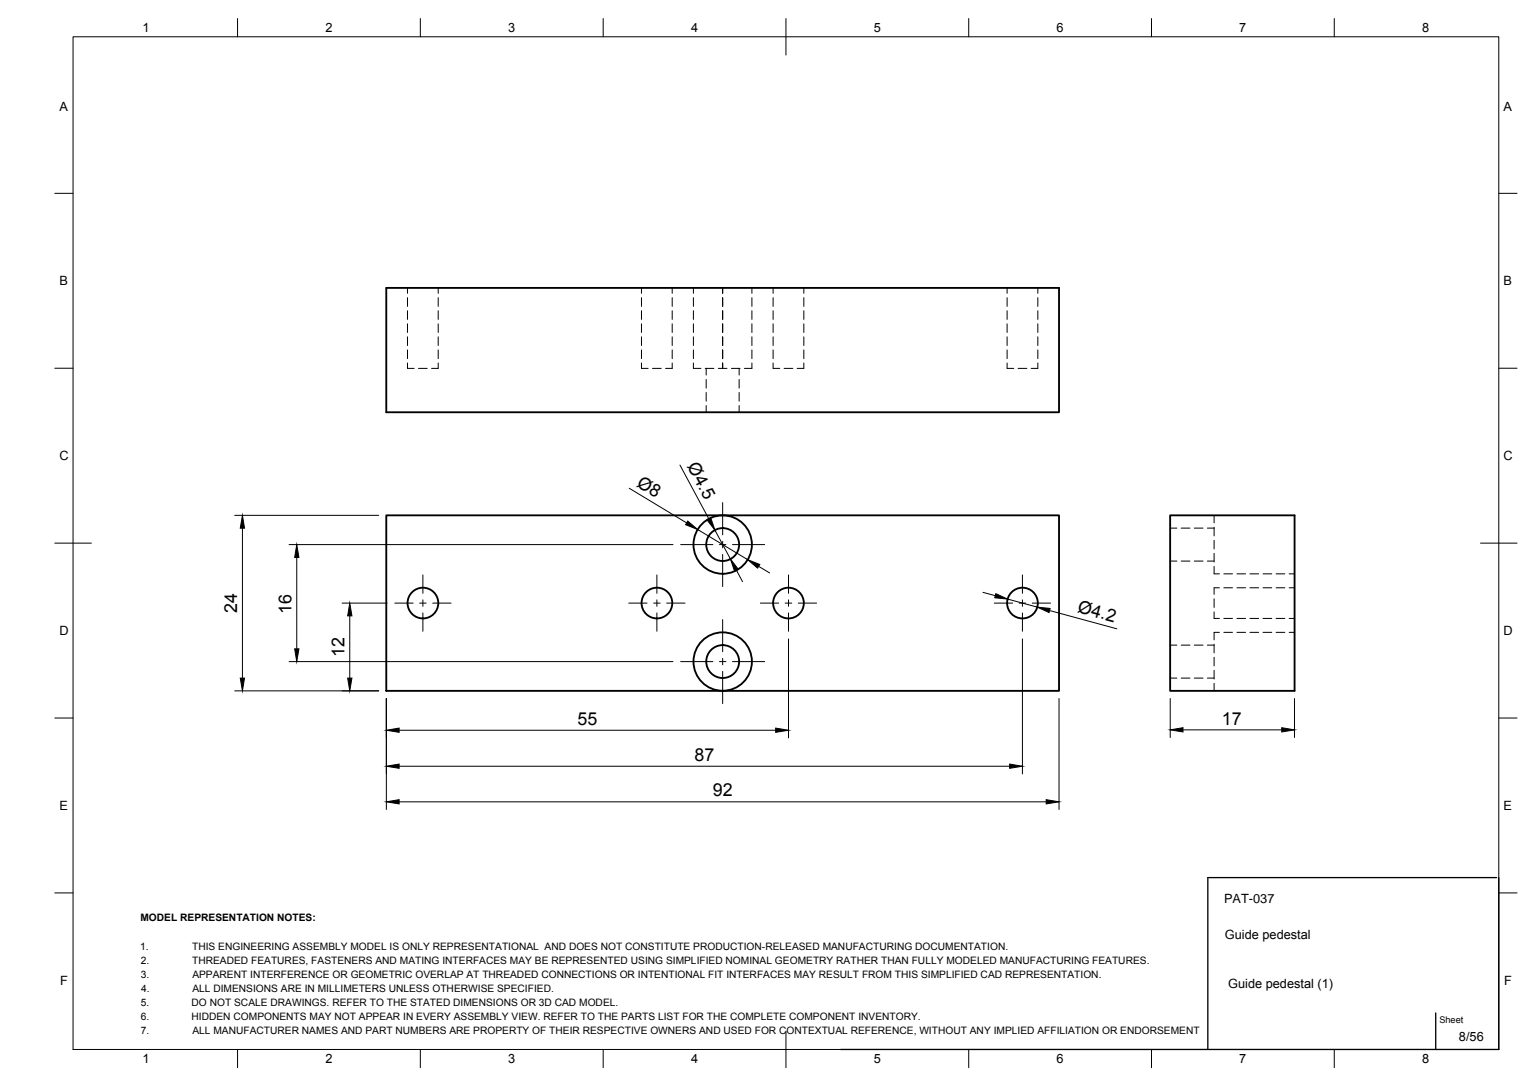
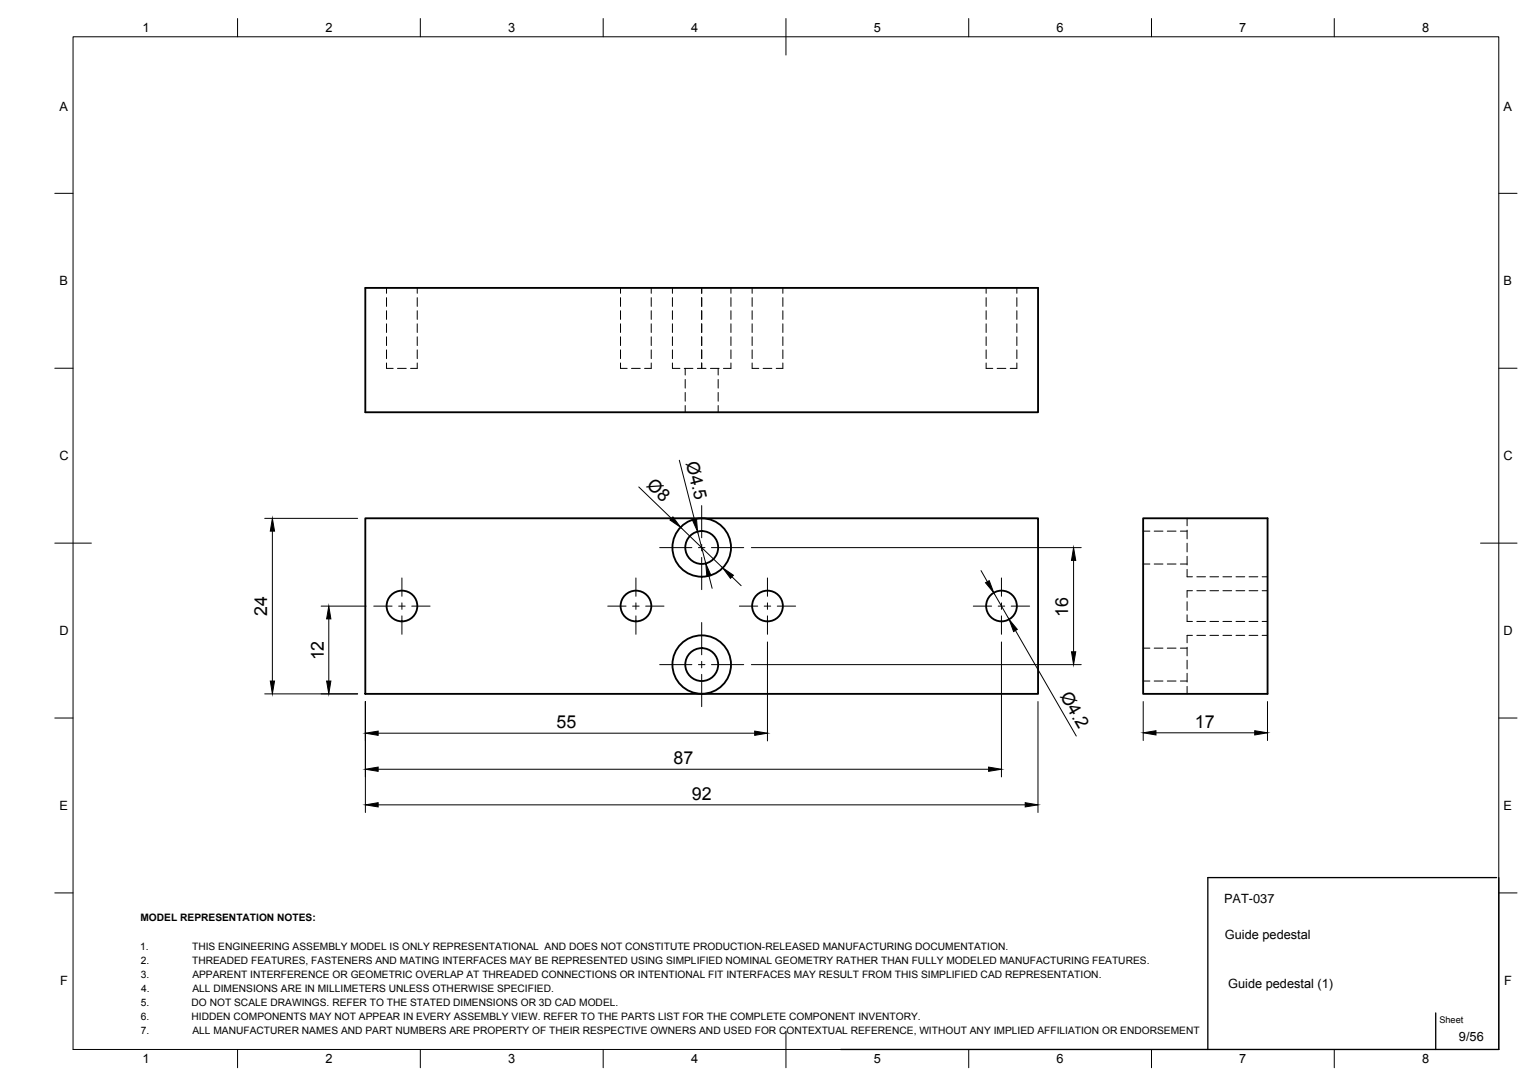
ISO-10303-21;
HEADER;
/* Generated by software containing ST-Developer
 * from STEP Tools, Inc. (www.steptools.com) 
 */

FILE_DESCRIPTION(
/* description */ ('Flywheel Crank-Slider'),
/* implementation_level */ '2;1');

FILE_NAME(
/* name */ 'Guide pedestal (1).step',
/* time_stamp */ '2026-10-28T03:23:13-07:00',
/* author */ (''),
/* organization */ (''),
/* preprocessor_version */ 'ST-DEVELOPER v20.2',
/* originating_system */ 'Autodesk Translation Framework v15.17.0.0',
/* authorisation */ '');

FILE_SCHEMA (('AUTOMOTIVE_DESIGN { 1 0 10303 214 3 1 1 }'));
ENDSEC;

DATA;
#10=MECHANICAL_DESIGN_GEOMETRIC_PRESENTATION_REPRESENTATION('',(#676),#17322);
#572=SHAPE_REPRESENTATION_RELATIONSHIP('SRR','None',#17568,#624);
#624=ADVANCED_BREP_SHAPE_REPRESENTATION('',(#737),#17272);
#676=STYLED_ITEM('',(#17945),#737);
#737=MANIFOLD_SOLID_BREP('Body1',#9054);
#853=FACE_BOUND('',#2025,.T.);
#854=FACE_BOUND('',#2028,.T.);
#855=FACE_BOUND('',#2030,.T.);
#856=FACE_BOUND('',#2031,.T.);
#857=FACE_BOUND('',#2032,.T.);
#858=FACE_BOUND('',#2033,.T.);
#859=FACE_BOUND('',#2049,.T.);
#860=FACE_BOUND('',#2050,.T.);
#1061=PLANE('',#9899);
#1062=PLANE('',#9904);
#1063=PLANE('',#9906);
#1064=PLANE('',#9917);
#1065=PLANE('',#9920);
#1066=PLANE('',#9923);
#1067=PLANE('',#9926);
#1068=PLANE('',#9927);
#1069=PLANE('',#9928);
#1070=PLANE('',#9929);
#1071=PLANE('',#9930);
#1072=PLANE('',#9931);
#1419=FACE_OUTER_BOUND('',#2022,.T.);
#1420=FACE_OUTER_BOUND('',#2023,.T.);
#1421=FACE_OUTER_BOUND('',#2024,.T.);
#1422=FACE_OUTER_BOUND('',#2026,.T.);
#1423=FACE_OUTER_BOUND('',#2027,.T.);
#1424=FACE_OUTER_BOUND('',#2029,.T.);
#1425=FACE_OUTER_BOUND('',#2034,.T.);
#1426=FACE_OUTER_BOUND('',#2035,.T.);
#1427=FACE_OUTER_BOUND('',#2036,.T.);
#1428=FACE_OUTER_BOUND('',#2037,.T.);
#1429=FACE_OUTER_BOUND('',#2038,.T.);
#1430=FACE_OUTER_BOUND('',#2039,.T.);
#1431=FACE_OUTER_BOUND('',#2040,.T.);
#1432=FACE_OUTER_BOUND('',#2041,.T.);
#1433=FACE_OUTER_BOUND('',#2042,.T.);
#1434=FACE_OUTER_BOUND('',#2043,.T.);
#1435=FACE_OUTER_BOUND('',#2044,.T.);
#1436=FACE_OUTER_BOUND('',#2045,.T.);
#1437=FACE_OUTER_BOUND('',#2046,.T.);
#1438=FACE_OUTER_BOUND('',#2047,.T.);
#1439=FACE_OUTER_BOUND('',#2048,.T.);
#2022=EDGE_LOOP('',(#6520,#6521,#6522,#6523));
#2023=EDGE_LOOP('',(#6524,#6525,#6526,#6527));
#2024=EDGE_LOOP('',(#6528));
#2025=EDGE_LOOP('',(#6529));
#2026=EDGE_LOOP('',(#6530,#6531,#6532,#6533));
#2027=EDGE_LOOP('',(#6534,#6535));
#2028=EDGE_LOOP('',(#6536));
#2029=EDGE_LOOP('',(#6537,#6538,#6539,#6540,#6541,#6542,#6543,#6544,#6545));
#2030=EDGE_LOOP('',(#6546));
#2031=EDGE_LOOP('',(#6547));
#2032=EDGE_LOOP('',(#6548));
#2033=EDGE_LOOP('',(#6549));
#2034=EDGE_LOOP('',(#6550,#6551,#6552,#6553));
#2035=EDGE_LOOP('',(#6554,#6555,#6556,#6557));
#2036=EDGE_LOOP('',(#6558,#6559,#6560,#6561));
#2037=EDGE_LOOP('',(#6562));
#2038=EDGE_LOOP('',(#6563,#6564,#6565,#6566));
#2039=EDGE_LOOP('',(#6567));
#2040=EDGE_LOOP('',(#6568,#6569,#6570,#6571));
#2041=EDGE_LOOP('',(#6572));
#2042=EDGE_LOOP('',(#6573,#6574,#6575,#6576));
#2043=EDGE_LOOP('',(#6577));
#2044=EDGE_LOOP('',(#6578,#6579,#6580,#6581));
#2045=EDGE_LOOP('',(#6582,#6583,#6584,#6585,#6586,#6587,#6588));
#2046=EDGE_LOOP('',(#6589,#6590,#6591,#6592));
#2047=EDGE_LOOP('',(#6593,#6594,#6595,#6596,#6597,#6598,#6599));
#2048=EDGE_LOOP('',(#6600,#6601,#6602,#6603));
#2049=EDGE_LOOP('',(#6604));
#2050=EDGE_LOOP('',(#6605));
#2717=LINE('',#14173,#3328);
#2718=LINE('',#14177,#3329);
#2719=LINE('',#14183,#3330);
#2720=LINE('',#14185,#3331);
#2721=LINE('',#14191,#3332);
#2722=LINE('',#14198,#3333);
#2723=LINE('',#14200,#3334);
#2724=LINE('',#14202,#3335);
#2725=LINE('',#14203,#3336);
#2726=LINE('',#14205,#3337);
#2727=LINE('',#14206,#3338);
#2728=LINE('',#14218,#3339);
#2729=LINE('',#14222,#3340);
#2730=LINE('',#14226,#3341);
#2731=LINE('',#14231,#3342);
#2732=LINE('',#14236,#3343);
#2733=LINE('',#14241,#3344);
#2734=LINE('',#14246,#3345);
#2735=LINE('',#14247,#3346);
#2736=LINE('',#14248,#3347);
#2737=LINE('',#14251,#3348);
#2738=LINE('',#14252,#3349);
#2739=LINE('',#14255,#3350);
#2740=LINE('',#14256,#3351);
#2741=LINE('',#14258,#3352);
#3328=VECTOR('',#11349,0.399999999999999);
#3329=VECTOR('',#11352,1.);
#3330=VECTOR('',#11359,1.);
#3331=VECTOR('',#11362,1.);
#3332=VECTOR('',#11371,1.);
#3333=VECTOR('',#11380,1.);
#3334=VECTOR('',#11381,1.);
#3335=VECTOR('',#11382,1.);
#3336=VECTOR('',#11383,1.);
#3337=VECTOR('',#11384,1.);
#3338=VECTOR('',#11385,1.);
#3339=VECTOR('',#11398,0.225000000000001);
#3340=VECTOR('',#11403,0.225000000000001);
#3341=VECTOR('',#11408,0.210000000000001);
#3342=VECTOR('',#11415,0.210000000000001);
#3343=VECTOR('',#11422,0.210000000000001);
#3344=VECTOR('',#11429,0.210000000000001);
#3345=VECTOR('',#11434,1.);
#3346=VECTOR('',#11435,1.);
#3347=VECTOR('',#11436,1.);
#3348=VECTOR('',#11439,1.);
#3349=VECTOR('',#11440,1.);
#3350=VECTOR('',#11443,1.);
#3351=VECTOR('',#11444,1.);
#3352=VECTOR('',#11447,1.);
#3936=CIRCLE('',#9894,0.399999999999999);
#3937=CIRCLE('',#9895,0.399999999999999);
#3938=CIRCLE('',#9897,0.399999999999999);
#3939=CIRCLE('',#9898,0.399999999999999);
#3940=CIRCLE('',#9900,0.225000000000001);
#3941=CIRCLE('',#9902,0.399999999999999);
#3942=CIRCLE('',#9903,0.399999999999999);
#3943=CIRCLE('',#9905,0.225000000000001);
#3944=CIRCLE('',#9907,0.210000000000001);
#3945=CIRCLE('',#9908,0.210000000000001);
#3946=CIRCLE('',#9909,0.210000000000001);
#3947=CIRCLE('',#9910,0.210000000000001);
#3948=CIRCLE('',#9912,0.225000000000001);
#3949=CIRCLE('',#9914,0.225000000000001);
#3950=CIRCLE('',#9916,0.210000000000001);
#3951=CIRCLE('',#9919,0.210000000000001);
#3952=CIRCLE('',#9922,0.210000000000001);
#3953=CIRCLE('',#9925,0.210000000000001);
#4407=VERTEX_POINT('',#14171);
#4408=VERTEX_POINT('',#14172);
#4409=VERTEX_POINT('',#14174);
#4410=VERTEX_POINT('',#14176);
#4411=VERTEX_POINT('',#14180);
#4412=VERTEX_POINT('',#14182);
#4413=VERTEX_POINT('',#14187);
#4414=VERTEX_POINT('',#14194);
#4415=VERTEX_POINT('',#14197);
#4416=VERTEX_POINT('',#14199);
#4417=VERTEX_POINT('',#14201);
#4418=VERTEX_POINT('',#14204);
#4419=VERTEX_POINT('',#14207);
#4420=VERTEX_POINT('',#14209);
#4421=VERTEX_POINT('',#14211);
#4422=VERTEX_POINT('',#14213);
#4423=VERTEX_POINT('',#14216);
#4424=VERTEX_POINT('',#14220);
#4425=VERTEX_POINT('',#14224);
#4426=VERTEX_POINT('',#14229);
#4427=VERTEX_POINT('',#14234);
#4428=VERTEX_POINT('',#14239);
#4429=VERTEX_POINT('',#14244);
#4430=VERTEX_POINT('',#14245);
#4431=VERTEX_POINT('',#14250);
#4432=VERTEX_POINT('',#14254);
#5217=EDGE_CURVE('',#4407,#4408,#2717,.T.);
#5218=EDGE_CURVE('',#4409,#4407,#3936,.T.);
#5219=EDGE_CURVE('',#4409,#4410,#2718,.T.);
#5220=EDGE_CURVE('',#4408,#4410,#3937,.T.);
#5221=EDGE_CURVE('',#4411,#4411,#3938,.T.);
#5222=EDGE_CURVE('',#4411,#4412,#2719,.T.);
#5223=EDGE_CURVE('',#4412,#4412,#3939,.T.);
#5224=EDGE_CURVE('',#4411,#4412,#2720,.T.);
#5225=EDGE_CURVE('',#4413,#4413,#3940,.T.);
#5226=EDGE_CURVE('',#4410,#4408,#3941,.T.);
#5227=EDGE_CURVE('',#4409,#4410,#2721,.T.);
#5228=EDGE_CURVE('',#4407,#4409,#3942,.T.);
#5229=EDGE_CURVE('',#4414,#4414,#3943,.T.);
#5230=EDGE_CURVE('',#4415,#4412,#2722,.T.);
#5231=EDGE_CURVE('',#4412,#4416,#2723,.T.);
#5232=EDGE_CURVE('',#4416,#4417,#2724,.T.);
#5233=EDGE_CURVE('',#4417,#4410,#2725,.T.);
#5234=EDGE_CURVE('',#4410,#4418,#2726,.T.);
#5235=EDGE_CURVE('',#4418,#4415,#2727,.T.);
#5236=EDGE_CURVE('',#4419,#4419,#3944,.T.);
#5237=EDGE_CURVE('',#4420,#4420,#3945,.T.);
#5238=EDGE_CURVE('',#4421,#4421,#3946,.T.);
#5239=EDGE_CURVE('',#4422,#4422,#3947,.T.);
#5240=EDGE_CURVE('',#4423,#4423,#3948,.T.);
#5241=EDGE_CURVE('',#4423,#4413,#2728,.T.);
#5242=EDGE_CURVE('',#4424,#4424,#3949,.T.);
#5243=EDGE_CURVE('',#4424,#4414,#2729,.T.);
#5244=EDGE_CURVE('',#4425,#4425,#3950,.T.);
#5245=EDGE_CURVE('',#4425,#4422,#2730,.T.);
#5246=EDGE_CURVE('',#4426,#4426,#3951,.T.);
#5247=EDGE_CURVE('',#4426,#4421,#2731,.T.);
#5248=EDGE_CURVE('',#4427,#4427,#3952,.T.);
#5249=EDGE_CURVE('',#4427,#4420,#2732,.T.);
#5250=EDGE_CURVE('',#4428,#4428,#3953,.T.);
#5251=EDGE_CURVE('',#4428,#4419,#2733,.T.);
#5252=EDGE_CURVE('',#4429,#4430,#2734,.T.);
#5253=EDGE_CURVE('',#4430,#4415,#2735,.T.);
#5254=EDGE_CURVE('',#4429,#4418,#2736,.T.);
#5255=EDGE_CURVE('',#4431,#4429,#2737,.T.);
#5256=EDGE_CURVE('',#4431,#4417,#2738,.T.);
#5257=EDGE_CURVE('',#4432,#4431,#2739,.T.);
#5258=EDGE_CURVE('',#4432,#4416,#2740,.T.);
#5259=EDGE_CURVE('',#4430,#4432,#2741,.T.);
#6520=ORIENTED_EDGE('',*,*,#5217,.F.);
#6521=ORIENTED_EDGE('',*,*,#5218,.F.);
#6522=ORIENTED_EDGE('',*,*,#5219,.T.);
#6523=ORIENTED_EDGE('',*,*,#5220,.F.);
#6524=ORIENTED_EDGE('',*,*,#5221,.F.);
#6525=ORIENTED_EDGE('',*,*,#5222,.T.);
#6526=ORIENTED_EDGE('',*,*,#5223,.F.);
#6527=ORIENTED_EDGE('',*,*,#5224,.F.);
#6528=ORIENTED_EDGE('',*,*,#5221,.T.);
#6529=ORIENTED_EDGE('',*,*,#5225,.F.);
#6530=ORIENTED_EDGE('',*,*,#5217,.T.);
#6531=ORIENTED_EDGE('',*,*,#5226,.F.);
#6532=ORIENTED_EDGE('',*,*,#5227,.F.);
#6533=ORIENTED_EDGE('',*,*,#5228,.F.);
#6534=ORIENTED_EDGE('',*,*,#5218,.T.);
#6535=ORIENTED_EDGE('',*,*,#5228,.T.);
#6536=ORIENTED_EDGE('',*,*,#5229,.F.);
#6537=ORIENTED_EDGE('',*,*,#5230,.T.);
#6538=ORIENTED_EDGE('',*,*,#5223,.T.);
#6539=ORIENTED_EDGE('',*,*,#5231,.T.);
#6540=ORIENTED_EDGE('',*,*,#5232,.T.);
#6541=ORIENTED_EDGE('',*,*,#5233,.T.);
#6542=ORIENTED_EDGE('',*,*,#5226,.T.);
#6543=ORIENTED_EDGE('',*,*,#5220,.T.);
#6544=ORIENTED_EDGE('',*,*,#5234,.T.);
#6545=ORIENTED_EDGE('',*,*,#5235,.T.);
#6546=ORIENTED_EDGE('',*,*,#5236,.T.);
#6547=ORIENTED_EDGE('',*,*,#5237,.T.);
#6548=ORIENTED_EDGE('',*,*,#5238,.T.);
#6549=ORIENTED_EDGE('',*,*,#5239,.T.);
#6550=ORIENTED_EDGE('',*,*,#5240,.F.);
#6551=ORIENTED_EDGE('',*,*,#5241,.T.);
#6552=ORIENTED_EDGE('',*,*,#5225,.T.);
#6553=ORIENTED_EDGE('',*,*,#5241,.F.);
#6554=ORIENTED_EDGE('',*,*,#5242,.F.);
#6555=ORIENTED_EDGE('',*,*,#5243,.T.);
#6556=ORIENTED_EDGE('',*,*,#5229,.T.);
#6557=ORIENTED_EDGE('',*,*,#5243,.F.);
#6558=ORIENTED_EDGE('',*,*,#5244,.F.);
#6559=ORIENTED_EDGE('',*,*,#5245,.T.);
#6560=ORIENTED_EDGE('',*,*,#5239,.F.);
#6561=ORIENTED_EDGE('',*,*,#5245,.F.);
#6562=ORIENTED_EDGE('',*,*,#5244,.T.);
#6563=ORIENTED_EDGE('',*,*,#5246,.F.);
#6564=ORIENTED_EDGE('',*,*,#5247,.T.);
#6565=ORIENTED_EDGE('',*,*,#5238,.F.);
#6566=ORIENTED_EDGE('',*,*,#5247,.F.);
#6567=ORIENTED_EDGE('',*,*,#5246,.T.);
#6568=ORIENTED_EDGE('',*,*,#5248,.F.);
#6569=ORIENTED_EDGE('',*,*,#5249,.T.);
#6570=ORIENTED_EDGE('',*,*,#5237,.F.);
#6571=ORIENTED_EDGE('',*,*,#5249,.F.);
#6572=ORIENTED_EDGE('',*,*,#5248,.T.);
#6573=ORIENTED_EDGE('',*,*,#5250,.F.);
#6574=ORIENTED_EDGE('',*,*,#5251,.T.);
#6575=ORIENTED_EDGE('',*,*,#5236,.F.);
#6576=ORIENTED_EDGE('',*,*,#5251,.F.);
#6577=ORIENTED_EDGE('',*,*,#5250,.T.);
#6578=ORIENTED_EDGE('',*,*,#5252,.T.);
#6579=ORIENTED_EDGE('',*,*,#5253,.T.);
#6580=ORIENTED_EDGE('',*,*,#5235,.F.);
#6581=ORIENTED_EDGE('',*,*,#5254,.F.);
#6582=ORIENTED_EDGE('',*,*,#5255,.T.);
#6583=ORIENTED_EDGE('',*,*,#5254,.T.);
#6584=ORIENTED_EDGE('',*,*,#5234,.F.);
#6585=ORIENTED_EDGE('',*,*,#5219,.F.);
#6586=ORIENTED_EDGE('',*,*,#5227,.T.);
#6587=ORIENTED_EDGE('',*,*,#5233,.F.);
#6588=ORIENTED_EDGE('',*,*,#5256,.F.);
#6589=ORIENTED_EDGE('',*,*,#5257,.T.);
#6590=ORIENTED_EDGE('',*,*,#5256,.T.);
#6591=ORIENTED_EDGE('',*,*,#5232,.F.);
#6592=ORIENTED_EDGE('',*,*,#5258,.F.);
#6593=ORIENTED_EDGE('',*,*,#5259,.T.);
#6594=ORIENTED_EDGE('',*,*,#5258,.T.);
#6595=ORIENTED_EDGE('',*,*,#5231,.F.);
#6596=ORIENTED_EDGE('',*,*,#5222,.F.);
#6597=ORIENTED_EDGE('',*,*,#5224,.T.);
#6598=ORIENTED_EDGE('',*,*,#5230,.F.);
#6599=ORIENTED_EDGE('',*,*,#5253,.F.);
#6600=ORIENTED_EDGE('',*,*,#5259,.F.);
#6601=ORIENTED_EDGE('',*,*,#5252,.F.);
#6602=ORIENTED_EDGE('',*,*,#5255,.F.);
#6603=ORIENTED_EDGE('',*,*,#5257,.F.);
#6604=ORIENTED_EDGE('',*,*,#5240,.T.);
#6605=ORIENTED_EDGE('',*,*,#5242,.T.);
#8379=CYLINDRICAL_SURFACE('',#9893,0.399999999999999);
#8380=CYLINDRICAL_SURFACE('',#9896,0.399999999999999);
#8381=CYLINDRICAL_SURFACE('',#9901,0.399999999999999);
#8382=CYLINDRICAL_SURFACE('',#9911,0.225000000000001);
#8383=CYLINDRICAL_SURFACE('',#9913,0.225000000000001);
#8384=CYLINDRICAL_SURFACE('',#9915,0.210000000000001);
#8385=CYLINDRICAL_SURFACE('',#9918,0.210000000000001);
#8386=CYLINDRICAL_SURFACE('',#9921,0.210000000000001);
#8387=CYLINDRICAL_SURFACE('',#9924,0.210000000000001);
#8610=ADVANCED_FACE('',(#1419),#8379,.F.);
#8611=ADVANCED_FACE('',(#1420),#8380,.F.);
#8612=ADVANCED_FACE('',(#1421,#853),#1061,.T.);
#8613=ADVANCED_FACE('',(#1422),#8381,.F.);
#8614=ADVANCED_FACE('',(#1423,#854),#1062,.T.);
#8615=ADVANCED_FACE('',(#1424,#855,#856,#857,#858),#1063,.T.);
#8616=ADVANCED_FACE('',(#1425),#8382,.F.);
#8617=ADVANCED_FACE('',(#1426),#8383,.F.);
#8618=ADVANCED_FACE('',(#1427),#8384,.F.);
#8619=ADVANCED_FACE('',(#1428),#1064,.T.);
#8620=ADVANCED_FACE('',(#1429),#8385,.F.);
#8621=ADVANCED_FACE('',(#1430),#1065,.T.);
#8622=ADVANCED_FACE('',(#1431),#8386,.F.);
#8623=ADVANCED_FACE('',(#1432),#1066,.T.);
#8624=ADVANCED_FACE('',(#1433),#8387,.F.);
#8625=ADVANCED_FACE('',(#1434),#1067,.T.);
#8626=ADVANCED_FACE('',(#1435),#1068,.T.);
#8627=ADVANCED_FACE('',(#1436),#1069,.T.);
#8628=ADVANCED_FACE('',(#1437),#1070,.T.);
#8629=ADVANCED_FACE('',(#1438),#1071,.T.);
#8630=ADVANCED_FACE('',(#1439,#859,#860),#1072,.F.);
#9054=CLOSED_SHELL('',(#8610,#8611,#8612,#8613,#8614,#8615,#8616,#8617,
#8618,#8619,#8620,#8621,#8622,#8623,#8624,#8625,#8626,#8627,#8628,#8629,
#8630));
#9892=AXIS2_PLACEMENT_3D('',#14169,#11345,#11346);
#9893=AXIS2_PLACEMENT_3D('',#14170,#11347,#11348);
#9894=AXIS2_PLACEMENT_3D('',#14175,#11350,#11351);
#9895=AXIS2_PLACEMENT_3D('',#14178,#11353,#11354);
#9896=AXIS2_PLACEMENT_3D('',#14179,#11355,#11356);
#9897=AXIS2_PLACEMENT_3D('',#14181,#11357,#11358);
#9898=AXIS2_PLACEMENT_3D('',#14184,#11360,#11361);
#9899=AXIS2_PLACEMENT_3D('',#14186,#11363,#11364);
#9900=AXIS2_PLACEMENT_3D('',#14188,#11365,#11366);
#9901=AXIS2_PLACEMENT_3D('',#14189,#11367,#11368);
#9902=AXIS2_PLACEMENT_3D('',#14190,#11369,#11370);
#9903=AXIS2_PLACEMENT_3D('',#14192,#11372,#11373);
#9904=AXIS2_PLACEMENT_3D('',#14193,#11374,#11375);
#9905=AXIS2_PLACEMENT_3D('',#14195,#11376,#11377);
#9906=AXIS2_PLACEMENT_3D('',#14196,#11378,#11379);
#9907=AXIS2_PLACEMENT_3D('',#14208,#11386,#11387);
#9908=AXIS2_PLACEMENT_3D('',#14210,#11388,#11389);
#9909=AXIS2_PLACEMENT_3D('',#14212,#11390,#11391);
#9910=AXIS2_PLACEMENT_3D('',#14214,#11392,#11393);
#9911=AXIS2_PLACEMENT_3D('',#14215,#11394,#11395);
#9912=AXIS2_PLACEMENT_3D('',#14217,#11396,#11397);
#9913=AXIS2_PLACEMENT_3D('',#14219,#11399,#11400);
#9914=AXIS2_PLACEMENT_3D('',#14221,#11401,#11402);
#9915=AXIS2_PLACEMENT_3D('',#14223,#11404,#11405);
#9916=AXIS2_PLACEMENT_3D('',#14225,#11406,#11407);
#9917=AXIS2_PLACEMENT_3D('',#14227,#11409,#11410);
#9918=AXIS2_PLACEMENT_3D('',#14228,#11411,#11412);
#9919=AXIS2_PLACEMENT_3D('',#14230,#11413,#11414);
#9920=AXIS2_PLACEMENT_3D('',#14232,#11416,#11417);
#9921=AXIS2_PLACEMENT_3D('',#14233,#11418,#11419);
#9922=AXIS2_PLACEMENT_3D('',#14235,#11420,#11421);
#9923=AXIS2_PLACEMENT_3D('',#14237,#11423,#11424);
#9924=AXIS2_PLACEMENT_3D('',#14238,#11425,#11426);
#9925=AXIS2_PLACEMENT_3D('',#14240,#11427,#11428);
#9926=AXIS2_PLACEMENT_3D('',#14242,#11430,#11431);
#9927=AXIS2_PLACEMENT_3D('',#14243,#11432,#11433);
#9928=AXIS2_PLACEMENT_3D('',#14249,#11437,#11438);
#9929=AXIS2_PLACEMENT_3D('',#14253,#11441,#11442);
#9930=AXIS2_PLACEMENT_3D('',#14257,#11445,#11446);
#9931=AXIS2_PLACEMENT_3D('',#14259,#11448,#11449);
#11345=DIRECTION('axis',(0.,0.,1.));
#11346=DIRECTION('refdir',(1.,0.,0.));
#11347=DIRECTION('center_axis',(0.,0.,1.));
#11348=DIRECTION('ref_axis',(1.,0.,0.));
#11349=DIRECTION('',(0.,0.,1.));
#11350=DIRECTION('center_axis',(0.,0.,1.));
#11351=DIRECTION('ref_axis',(1.,0.,0.));
#11352=DIRECTION('',(0.,0.,1.));
#11353=DIRECTION('center_axis',(0.,0.,-1.));
#11354=DIRECTION('ref_axis',(1.,0.,0.));
#11355=DIRECTION('center_axis',(0.,0.,1.));
#11356=DIRECTION('ref_axis',(1.,0.,0.));
#11357=DIRECTION('center_axis',(0.,0.,1.));
#11358=DIRECTION('ref_axis',(1.,0.,0.));
#11359=DIRECTION('',(0.,0.,1.));
#11360=DIRECTION('center_axis',(0.,0.,-1.));
#11361=DIRECTION('ref_axis',(1.,0.,0.));
#11362=DIRECTION('',(0.,0.,1.));
#11363=DIRECTION('center_axis',(0.,0.,1.));
#11364=DIRECTION('ref_axis',(1.,0.,0.));
#11365=DIRECTION('center_axis',(0.,0.,1.));
#11366=DIRECTION('ref_axis',(1.,0.,0.));
#11367=DIRECTION('center_axis',(0.,0.,1.));
#11368=DIRECTION('ref_axis',(1.,0.,0.));
#11369=DIRECTION('center_axis',(0.,0.,-1.));
#11370=DIRECTION('ref_axis',(1.,0.,0.));
#11371=DIRECTION('',(0.,0.,1.));
#11372=DIRECTION('center_axis',(0.,0.,1.));
#11373=DIRECTION('ref_axis',(1.,0.,0.));
#11374=DIRECTION('center_axis',(0.,0.,1.));
#11375=DIRECTION('ref_axis',(1.,0.,0.));
#11376=DIRECTION('center_axis',(0.,0.,1.));
#11377=DIRECTION('ref_axis',(1.,0.,0.));
#11378=DIRECTION('center_axis',(0.,0.,1.));
#11379=DIRECTION('ref_axis',(1.,0.,0.));
#11380=DIRECTION('',(0.,-1.,0.));
#11381=DIRECTION('',(0.,-1.,0.));
#11382=DIRECTION('',(1.,0.,0.));
#11383=DIRECTION('',(0.,1.,0.));
#11384=DIRECTION('',(0.,1.,0.));
#11385=DIRECTION('',(-1.,0.,0.));
#11386=DIRECTION('center_axis',(0.,0.,-1.));
#11387=DIRECTION('ref_axis',(1.,0.,0.));
#11388=DIRECTION('center_axis',(0.,0.,-1.));
#11389=DIRECTION('ref_axis',(1.,0.,0.));
#11390=DIRECTION('center_axis',(0.,0.,-1.));
#11391=DIRECTION('ref_axis',(1.,0.,0.));
#11392=DIRECTION('center_axis',(0.,0.,-1.));
#11393=DIRECTION('ref_axis',(1.,0.,0.));
#11394=DIRECTION('center_axis',(0.,0.,1.));
#11395=DIRECTION('ref_axis',(1.,0.,0.));
#11396=DIRECTION('center_axis',(0.,0.,1.));
#11397=DIRECTION('ref_axis',(1.,0.,0.));
#11398=DIRECTION('',(0.,0.,1.));
#11399=DIRECTION('center_axis',(0.,0.,1.));
#11400=DIRECTION('ref_axis',(1.,0.,0.));
#11401=DIRECTION('center_axis',(0.,0.,1.));
#11402=DIRECTION('ref_axis',(1.,0.,0.));
#11403=DIRECTION('',(0.,0.,1.));
#11404=DIRECTION('center_axis',(0.,0.,1.));
#11405=DIRECTION('ref_axis',(1.,0.,0.));
#11406=DIRECTION('center_axis',(0.,0.,1.));
#11407=DIRECTION('ref_axis',(1.,0.,0.));
#11408=DIRECTION('',(0.,0.,1.));
#11409=DIRECTION('center_axis',(0.,0.,1.));
#11410=DIRECTION('ref_axis',(1.,0.,0.));
#11411=DIRECTION('center_axis',(0.,0.,1.));
#11412=DIRECTION('ref_axis',(1.,0.,0.));
#11413=DIRECTION('center_axis',(0.,0.,1.));
#11414=DIRECTION('ref_axis',(1.,0.,0.));
#11415=DIRECTION('',(0.,0.,1.));
#11416=DIRECTION('center_axis',(0.,0.,1.));
#11417=DIRECTION('ref_axis',(1.,0.,0.));
#11418=DIRECTION('center_axis',(0.,0.,1.));
#11419=DIRECTION('ref_axis',(1.,0.,0.));
#11420=DIRECTION('center_axis',(0.,0.,1.));
#11421=DIRECTION('ref_axis',(1.,0.,0.));
#11422=DIRECTION('',(0.,0.,1.));
#11423=DIRECTION('center_axis',(0.,0.,1.));
#11424=DIRECTION('ref_axis',(1.,0.,0.));
#11425=DIRECTION('center_axis',(0.,0.,1.));
#11426=DIRECTION('ref_axis',(1.,0.,0.));
#11427=DIRECTION('center_axis',(0.,0.,1.));
#11428=DIRECTION('ref_axis',(1.,0.,0.));
#11429=DIRECTION('',(0.,0.,1.));
#11430=DIRECTION('center_axis',(0.,0.,1.));
#11431=DIRECTION('ref_axis',(1.,0.,0.));
#11432=DIRECTION('center_axis',(0.,1.,0.));
#11433=DIRECTION('ref_axis',(-1.,0.,0.));
#11434=DIRECTION('',(-1.,0.,0.));
#11435=DIRECTION('',(0.,0.,1.));
#11436=DIRECTION('',(0.,0.,1.));
#11437=DIRECTION('center_axis',(1.,0.,0.));
#11438=DIRECTION('ref_axis',(0.,1.,0.));
#11439=DIRECTION('',(0.,1.,0.));
#11440=DIRECTION('',(0.,0.,1.));
#11441=DIRECTION('center_axis',(0.,-1.,0.));
#11442=DIRECTION('ref_axis',(1.,0.,0.));
#11443=DIRECTION('',(1.,0.,0.));
#11444=DIRECTION('',(0.,0.,1.));
#11445=DIRECTION('center_axis',(-1.,0.,0.));
#11446=DIRECTION('ref_axis',(0.,-1.,0.));
#11447=DIRECTION('',(0.,-1.,0.));
#11448=DIRECTION('center_axis',(0.,0.,1.));
#11449=DIRECTION('ref_axis',(1.,0.,0.));
#14169=CARTESIAN_POINT('',(0.,0.,0.));
#14170=CARTESIAN_POINT('Origin',(20.8,0.,1.6));
#14171=CARTESIAN_POINT('',(20.4,-4.8985871965894E-17,1.6));
#14172=CARTESIAN_POINT('',(20.4,-4.8985871965894E-17,2.7));
#14173=CARTESIAN_POINT('',(20.4,-4.8985871965894E-17,1.6));
#14174=CARTESIAN_POINT('',(21.2,0.,1.6));
#14175=CARTESIAN_POINT('Origin',(20.8,0.,1.6));
#14176=CARTESIAN_POINT('',(21.2,0.,2.7));
#14177=CARTESIAN_POINT('',(21.2,0.,1.6));
#14178=CARTESIAN_POINT('Origin',(20.8,0.,2.7));
#14179=CARTESIAN_POINT('Origin',(19.2,0.,1.6));
#14180=CARTESIAN_POINT('',(18.8,-4.8985871965894E-17,1.6));
#14181=CARTESIAN_POINT('Origin',(19.2,0.,1.6));
#14182=CARTESIAN_POINT('',(18.8,0.,2.7));
#14183=CARTESIAN_POINT('',(18.8,0.,1.6));
#14184=CARTESIAN_POINT('Origin',(19.2,0.,2.7));
#14185=CARTESIAN_POINT('',(18.8,0.,1.6));
#14186=CARTESIAN_POINT('Origin',(19.2,0.,1.6));
#14187=CARTESIAN_POINT('',(18.975,-2.75545529808156E-17,1.6));
#14188=CARTESIAN_POINT('Origin',(19.2,0.,1.6));
#14189=CARTESIAN_POINT('Origin',(20.8,0.,1.6));
#14190=CARTESIAN_POINT('Origin',(20.8,0.,2.7));
#14191=CARTESIAN_POINT('',(21.2,0.,1.6));
#14192=CARTESIAN_POINT('Origin',(20.8,0.,1.6));
#14193=CARTESIAN_POINT('Origin',(20.8,0.,1.6));
#14194=CARTESIAN_POINT('',(20.575,-2.75545529808156E-17,1.6));
#14195=CARTESIAN_POINT('Origin',(20.8,0.,1.6));
#14196=CARTESIAN_POINT('Origin',(20.,0.,2.7));
#14197=CARTESIAN_POINT('',(18.8,4.6,2.7));
#14198=CARTESIAN_POINT('',(18.8,4.6,2.7));
#14199=CARTESIAN_POINT('',(18.8,-4.6,2.7));
#14200=CARTESIAN_POINT('',(18.8,4.6,2.7));
#14201=CARTESIAN_POINT('',(21.2,-4.6,2.7));
#14202=CARTESIAN_POINT('',(18.8,-4.6,2.7));
#14203=CARTESIAN_POINT('',(21.2,-4.6,2.7));
#14204=CARTESIAN_POINT('',(21.2,4.6,2.7));
#14205=CARTESIAN_POINT('',(21.2,-4.6,2.7));
#14206=CARTESIAN_POINT('',(21.2,4.6,2.7));
#14207=CARTESIAN_POINT('',(19.79,4.1,2.7));
#14208=CARTESIAN_POINT('Origin',(20.,4.1,2.7));
#14209=CARTESIAN_POINT('',(19.79,-4.1,2.7));
#14210=CARTESIAN_POINT('Origin',(20.,-4.1,2.7));
#14211=CARTESIAN_POINT('',(19.79,-0.9,2.7));
#14212=CARTESIAN_POINT('Origin',(20.,-0.9,2.7));
#14213=CARTESIAN_POINT('',(19.79,0.9,2.7));
#14214=CARTESIAN_POINT('Origin',(20.,0.9,2.7));
#14215=CARTESIAN_POINT('Origin',(19.2,0.,0.9));
#14216=CARTESIAN_POINT('',(18.975,-2.75545529808156E-17,1.));
#14217=CARTESIAN_POINT('Origin',(19.2,0.,1.));
#14218=CARTESIAN_POINT('',(18.975,-2.75545529808156E-17,0.9));
#14219=CARTESIAN_POINT('Origin',(20.8,0.,0.9));
#14220=CARTESIAN_POINT('',(20.575,-2.75545529808156E-17,1.));
#14221=CARTESIAN_POINT('Origin',(20.8,0.,1.));
#14222=CARTESIAN_POINT('',(20.575,-2.75545529808156E-17,0.9));
#14223=CARTESIAN_POINT('Origin',(20.,0.9,1.6));
#14224=CARTESIAN_POINT('',(19.79,0.9,1.6));
#14225=CARTESIAN_POINT('Origin',(20.,0.9,1.6));
#14226=CARTESIAN_POINT('',(19.79,0.9,1.6));
#14227=CARTESIAN_POINT('Origin',(20.,0.9,1.6));
#14228=CARTESIAN_POINT('Origin',(20.,-0.9,1.6));
#14229=CARTESIAN_POINT('',(19.79,-0.9,1.6));
#14230=CARTESIAN_POINT('Origin',(20.,-0.9,1.6));
#14231=CARTESIAN_POINT('',(19.79,-0.9,1.6));
#14232=CARTESIAN_POINT('Origin',(20.,-0.9,1.6));
#14233=CARTESIAN_POINT('Origin',(20.,-4.1,1.6));
#14234=CARTESIAN_POINT('',(19.79,-4.1,1.6));
#14235=CARTESIAN_POINT('Origin',(20.,-4.1,1.6));
#14236=CARTESIAN_POINT('',(19.79,-4.1,1.6));
#14237=CARTESIAN_POINT('Origin',(20.,-4.1,1.6));
#14238=CARTESIAN_POINT('Origin',(20.,4.1,1.6));
#14239=CARTESIAN_POINT('',(19.79,4.1,1.6));
#14240=CARTESIAN_POINT('Origin',(20.,4.1,1.6));
#14241=CARTESIAN_POINT('',(19.79,4.1,1.6));
#14242=CARTESIAN_POINT('Origin',(20.,4.1,1.6));
#14243=CARTESIAN_POINT('Origin',(21.2,4.6,1.));
#14244=CARTESIAN_POINT('',(21.2,4.6,1.));
#14245=CARTESIAN_POINT('',(18.8,4.6,1.));
#14246=CARTESIAN_POINT('',(21.2,4.6,1.));
#14247=CARTESIAN_POINT('',(18.8,4.6,1.));
#14248=CARTESIAN_POINT('',(21.2,4.6,1.));
#14249=CARTESIAN_POINT('Origin',(21.2,-4.6,1.));
#14250=CARTESIAN_POINT('',(21.2,-4.6,1.));
#14251=CARTESIAN_POINT('',(21.2,-4.6,1.));
#14252=CARTESIAN_POINT('',(21.2,-4.6,1.));
#14253=CARTESIAN_POINT('Origin',(18.8,-4.6,1.));
#14254=CARTESIAN_POINT('',(18.8,-4.6,1.));
#14255=CARTESIAN_POINT('',(18.8,-4.6,1.));
#14256=CARTESIAN_POINT('',(18.8,-4.6,1.));
#14257=CARTESIAN_POINT('Origin',(18.8,4.6,1.));
#14258=CARTESIAN_POINT('',(18.8,4.6,1.));
#14259=CARTESIAN_POINT('Origin',(20.,0.,1.));
#17211=UNCERTAINTY_MEASURE_WITH_UNIT(LENGTH_MEASURE(0.001),#17323,
'DISTANCE_ACCURACY_VALUE',
'Maximum model space distance between geometric entities at asserted c
onnectivities');
#17261=UNCERTAINTY_MEASURE_WITH_UNIT(LENGTH_MEASURE(0.001),#17323,
'DISTANCE_ACCURACY_VALUE',
'Maximum model space distance between geometric entities at asserted c
onnectivities');
#17272=(
GEOMETRIC_REPRESENTATION_CONTEXT(3)
GLOBAL_UNCERTAINTY_ASSIGNED_CONTEXT((#17211))
GLOBAL_UNIT_ASSIGNED_CONTEXT((#17323,#17325,#17326))
REPRESENTATION_CONTEXT('','3D')
);
#17322=(
GEOMETRIC_REPRESENTATION_CONTEXT(3)
GLOBAL_UNCERTAINTY_ASSIGNED_CONTEXT((#17261))
GLOBAL_UNIT_ASSIGNED_CONTEXT((#17323,#17325,#17326))
REPRESENTATION_CONTEXT('','3D')
);
#17323=(
LENGTH_UNIT()
NAMED_UNIT(*)
SI_UNIT(.CENTI.,.METRE.)
);
#17325=(
NAMED_UNIT(*)
PLANE_ANGLE_UNIT()
SI_UNIT($,.RADIAN.)
);
#17326=(
NAMED_UNIT(*)
SI_UNIT($,.STERADIAN.)
SOLID_ANGLE_UNIT()
);
#17337=SHAPE_DEFINITION_REPRESENTATION(#17397,#17568);
#17397=PRODUCT_DEFINITION_SHAPE('',$,#17629);
#17568=SHAPE_REPRESENTATION('',(#9892),#17272);
#17618=PRODUCT_DEFINITION_CONTEXT('part definition',#17800,'design');
#17629=PRODUCT_DEFINITION('Guide pedestal (1)','Guide pedestal (1)',#17689,
#17618);
#17689=PRODUCT_DEFINITION_FORMATION('',$,#17812);
#17800=APPLICATION_CONTEXT(
'Core Data for Automotive Mechanical Design Process');
#17801=PRODUCT_CONTEXT('part definition',#17800,'mechanical');
#17812=PRODUCT('Guide pedestal (1)','Guide pedestal (1)','Guide pedestal (1)',
(#17801));
#17939=COLOUR_RGB('Off White',0.89,0.88,0.83);
#17940=FILL_AREA_STYLE_COLOUR('',#17939);
#17941=FILL_AREA_STYLE('',(#17940));
#17942=SURFACE_STYLE_FILL_AREA(#17941);
#17943=SURFACE_SIDE_STYLE('',(#17942));
#17944=SURFACE_STYLE_USAGE(.BOTH.,#17943);
#17945=PRESENTATION_STYLE_ASSIGNMENT((#17944));
ENDSEC;
END-ISO-10303-21;
